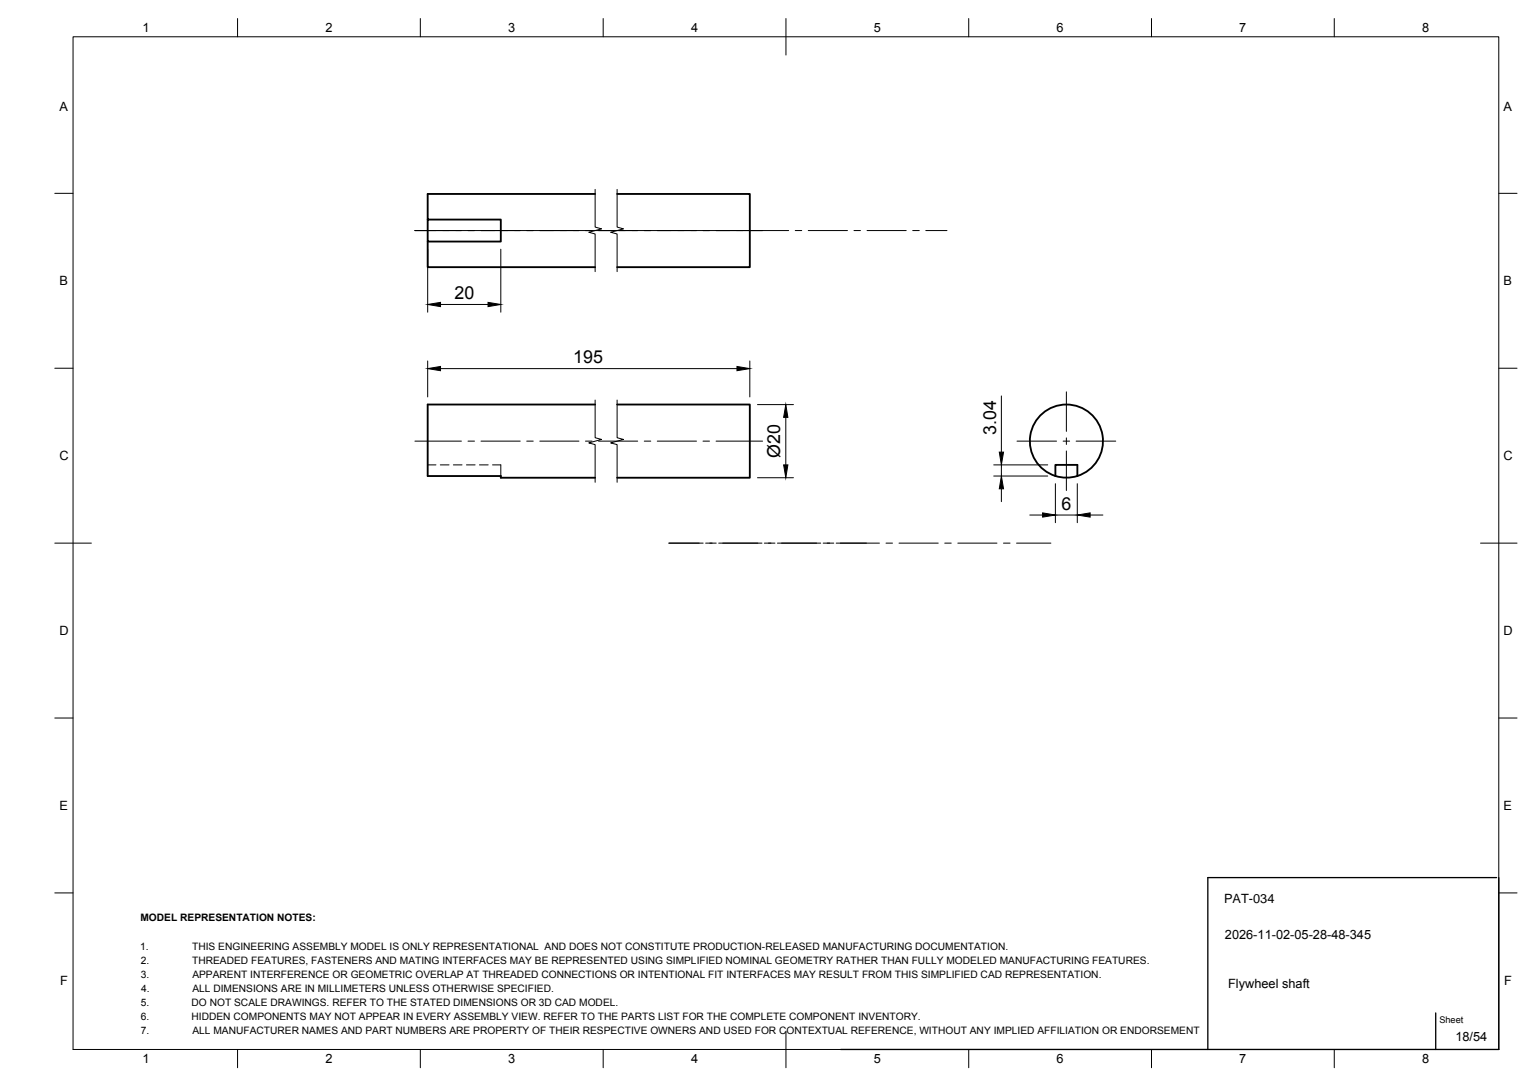
ISO-10303-21;
HEADER;
/* Generated by software containing ST-Developer
 * from STEP Tools, Inc. (www.steptools.com) 
 */

FILE_DESCRIPTION(
/* description */ ('Fatigue rig crank-slider'),
/* implementation_level */ '2;1');

FILE_NAME(
/* name */ 'Flywheel shaft.step',
/* time_stamp */ '2026-10-28T03:24:50-07:00',
/* author */ (''),
/* organization */ (''),
/* preprocessor_version */ 'ST-DEVELOPER v20.2',
/* originating_system */ 'Autodesk Translation Framework v15.17.0.0',
/* authorisation */ '');

FILE_SCHEMA (('AUTOMOTIVE_DESIGN { 1 0 10303 214 3 1 1 }'));
ENDSEC;

DATA;
#10=MECHANICAL_DESIGN_GEOMETRIC_PRESENTATION_REPRESENTATION('',(#604),#16911);
#503=SHAPE_REPRESENTATION_RELATIONSHIP('SRR','None',#17144,#553);
#553=ADVANCED_BREP_SHAPE_REPRESENTATION('',(#661),#16873);
#604=STYLED_ITEM('',(#17487),#661);
#661=MANIFOLD_SOLID_BREP('Body1',#8897);
#1027=PLANE('',#9901);
#1028=PLANE('',#9902);
#1029=PLANE('',#9904);
#1030=PLANE('',#9905);
#1031=PLANE('',#9910);
#1032=PLANE('',#9911);
#1437=FACE_OUTER_BOUND('',#2081,.T.);
#1438=FACE_OUTER_BOUND('',#2082,.T.);
#1439=FACE_OUTER_BOUND('',#2083,.T.);
#1440=FACE_OUTER_BOUND('',#2084,.T.);
#1441=FACE_OUTER_BOUND('',#2085,.T.);
#1442=FACE_OUTER_BOUND('',#2086,.T.);
#1443=FACE_OUTER_BOUND('',#2087,.T.);
#2081=EDGE_LOOP('',(#6920,#6921,#6922,#6923));
#2082=EDGE_LOOP('',(#6924,#6925,#6926,#6927));
#2083=EDGE_LOOP('',(#6928,#6929,#6930,#6931));
#2084=EDGE_LOOP('',(#6932,#6933,#6934,#6935));
#2085=EDGE_LOOP('',(#6936,#6937,#6938,#6939,#6940,#6941,#6942,#6943));
#2086=EDGE_LOOP('',(#6944,#6945,#6946,#6947,#6948));
#2087=EDGE_LOOP('',(#6949));
#2733=LINE('',#14787,#3379);
#2734=LINE('',#14789,#3380);
#2735=LINE('',#14791,#3381);
#2736=LINE('',#14792,#3382);
#2737=LINE('',#14797,#3383);
#2738=LINE('',#14798,#3384);
#2739=LINE('',#14801,#3385);
#2740=LINE('',#14803,#3386);
#2741=LINE('',#14804,#3387);
#2742=LINE('',#14806,#3388);
#2743=LINE('',#14811,#3389);
#3379=VECTOR('',#11657,1.);
#3380=VECTOR('',#11658,1.);
#3381=VECTOR('',#11659,1.);
#3382=VECTOR('',#11660,1.);
#3383=VECTOR('',#11665,1.);
#3384=VECTOR('',#11666,1.);
#3385=VECTOR('',#11669,1.);
#3386=VECTOR('',#11670,1.);
#3387=VECTOR('',#11671,1.);
#3388=VECTOR('',#11674,1.);
#3389=VECTOR('',#11679,1.);
#3917=CIRCLE('',#9903,1.);
#3918=CIRCLE('',#9907,1.);
#3919=CIRCLE('',#9908,1.);
#3920=CIRCLE('',#9909,1.);
#4465=VERTEX_POINT('',#14785);
#4466=VERTEX_POINT('',#14786);
#4467=VERTEX_POINT('',#14788);
#4468=VERTEX_POINT('',#14790);
#4469=VERTEX_POINT('',#14794);
#4470=VERTEX_POINT('',#14796);
#4471=VERTEX_POINT('',#14800);
#4472=VERTEX_POINT('',#14802);
#4473=VERTEX_POINT('',#14808);
#4474=VERTEX_POINT('',#14810);
#5358=EDGE_CURVE('',#4465,#4466,#2733,.T.);
#5359=EDGE_CURVE('',#4467,#4465,#2734,.T.);
#5360=EDGE_CURVE('',#4468,#4467,#2735,.T.);
#5361=EDGE_CURVE('',#4468,#4466,#2736,.T.);
#5362=EDGE_CURVE('',#4466,#4469,#3917,.T.);
#5363=EDGE_CURVE('',#4470,#4468,#2737,.T.);
#5364=EDGE_CURVE('',#4469,#4470,#2738,.T.);
#5365=EDGE_CURVE('',#4469,#4471,#2739,.T.);
#5366=EDGE_CURVE('',#4470,#4472,#2740,.T.);
#5367=EDGE_CURVE('',#4471,#4472,#2741,.T.);
#5368=EDGE_CURVE('',#4472,#4467,#2742,.T.);
#5369=EDGE_CURVE('',#4473,#4471,#3918,.T.);
#5370=EDGE_CURVE('',#4473,#4474,#2743,.T.);
#5371=EDGE_CURVE('',#4474,#4474,#3919,.T.);
#5372=EDGE_CURVE('',#4465,#4473,#3920,.T.);
#6920=ORIENTED_EDGE('',*,*,#5358,.F.);
#6921=ORIENTED_EDGE('',*,*,#5359,.F.);
#6922=ORIENTED_EDGE('',*,*,#5360,.F.);
#6923=ORIENTED_EDGE('',*,*,#5361,.T.);
#6924=ORIENTED_EDGE('',*,*,#5362,.F.);
#6925=ORIENTED_EDGE('',*,*,#5361,.F.);
#6926=ORIENTED_EDGE('',*,*,#5363,.F.);
#6927=ORIENTED_EDGE('',*,*,#5364,.F.);
#6928=ORIENTED_EDGE('',*,*,#5365,.F.);
#6929=ORIENTED_EDGE('',*,*,#5364,.T.);
#6930=ORIENTED_EDGE('',*,*,#5366,.T.);
#6931=ORIENTED_EDGE('',*,*,#5367,.F.);
#6932=ORIENTED_EDGE('',*,*,#5363,.T.);
#6933=ORIENTED_EDGE('',*,*,#5360,.T.);
#6934=ORIENTED_EDGE('',*,*,#5368,.F.);
#6935=ORIENTED_EDGE('',*,*,#5366,.F.);
#6936=ORIENTED_EDGE('',*,*,#5358,.T.);
#6937=ORIENTED_EDGE('',*,*,#5362,.T.);
#6938=ORIENTED_EDGE('',*,*,#5365,.T.);
#6939=ORIENTED_EDGE('',*,*,#5369,.F.);
#6940=ORIENTED_EDGE('',*,*,#5370,.T.);
#6941=ORIENTED_EDGE('',*,*,#5371,.T.);
#6942=ORIENTED_EDGE('',*,*,#5370,.F.);
#6943=ORIENTED_EDGE('',*,*,#5372,.F.);
#6944=ORIENTED_EDGE('',*,*,#5359,.T.);
#6945=ORIENTED_EDGE('',*,*,#5372,.T.);
#6946=ORIENTED_EDGE('',*,*,#5369,.T.);
#6947=ORIENTED_EDGE('',*,*,#5367,.T.);
#6948=ORIENTED_EDGE('',*,*,#5368,.T.);
#6949=ORIENTED_EDGE('',*,*,#5371,.F.);
#8277=CYLINDRICAL_SURFACE('',#9906,1.);
#8575=ADVANCED_FACE('',(#1437),#1027,.F.);
#8576=ADVANCED_FACE('',(#1438),#1028,.T.);
#8577=ADVANCED_FACE('',(#1439),#1029,.F.);
#8578=ADVANCED_FACE('',(#1440),#1030,.F.);
#8579=ADVANCED_FACE('',(#1441),#8277,.T.);
#8580=ADVANCED_FACE('',(#1442),#1031,.T.);
#8581=ADVANCED_FACE('',(#1443),#1032,.F.);
#8897=CLOSED_SHELL('',(#8575,#8576,#8577,#8578,#8579,#8580,#8581));
#9900=AXIS2_PLACEMENT_3D('',#14783,#11653,#11654);
#9901=AXIS2_PLACEMENT_3D('',#14784,#11655,#11656);
#9902=AXIS2_PLACEMENT_3D('',#14793,#11661,#11662);
#9903=AXIS2_PLACEMENT_3D('',#14795,#11663,#11664);
#9904=AXIS2_PLACEMENT_3D('',#14799,#11667,#11668);
#9905=AXIS2_PLACEMENT_3D('',#14805,#11672,#11673);
#9906=AXIS2_PLACEMENT_3D('',#14807,#11675,#11676);
#9907=AXIS2_PLACEMENT_3D('',#14809,#11677,#11678);
#9908=AXIS2_PLACEMENT_3D('',#14812,#11680,#11681);
#9909=AXIS2_PLACEMENT_3D('',#14813,#11682,#11683);
#9910=AXIS2_PLACEMENT_3D('',#14814,#11684,#11685);
#9911=AXIS2_PLACEMENT_3D('',#14815,#11686,#11687);
#11653=DIRECTION('axis',(0.,0.,1.));
#11654=DIRECTION('refdir',(1.,0.,0.));
#11655=DIRECTION('center_axis',(-1.,0.,0.));
#11656=DIRECTION('ref_axis',(0.,0.,1.));
#11657=DIRECTION('',(0.,-1.,0.));
#11658=DIRECTION('',(0.,0.,-1.));
#11659=DIRECTION('',(0.,1.,0.));
#11660=DIRECTION('',(0.,0.,-1.));
#11661=DIRECTION('center_axis',(0.,1.,0.));
#11662=DIRECTION('ref_axis',(1.,0.,0.));
#11663=DIRECTION('center_axis',(0.,-1.,0.));
#11664=DIRECTION('ref_axis',(1.,0.,0.));
#11665=DIRECTION('',(-1.,0.,0.));
#11666=DIRECTION('',(0.,0.,1.));
#11667=DIRECTION('center_axis',(1.,0.,0.));
#11668=DIRECTION('ref_axis',(0.,0.,-1.));
#11669=DIRECTION('',(0.,1.,0.));
#11670=DIRECTION('',(0.,1.,0.));
#11671=DIRECTION('',(0.,0.,1.));
#11672=DIRECTION('center_axis',(0.,0.,1.));
#11673=DIRECTION('ref_axis',(1.,0.,0.));
#11674=DIRECTION('',(-1.,0.,0.));
#11675=DIRECTION('center_axis',(0.,1.,0.));
#11676=DIRECTION('ref_axis',(1.,0.,0.));
#11677=DIRECTION('center_axis',(0.,1.,0.));
#11678=DIRECTION('ref_axis',(1.,0.,0.));
#11679=DIRECTION('',(0.,-1.,0.));
#11680=DIRECTION('center_axis',(0.,1.,0.));
#11681=DIRECTION('ref_axis',(1.,0.,0.));
#11682=DIRECTION('center_axis',(0.,1.,0.));
#11683=DIRECTION('ref_axis',(1.,0.,0.));
#11684=DIRECTION('center_axis',(0.,1.,0.));
#11685=DIRECTION('ref_axis',(1.,0.,0.));
#11686=DIRECTION('center_axis',(0.,1.,0.));
#11687=DIRECTION('ref_axis',(1.,0.,0.));
#14783=CARTESIAN_POINT('',(0.,0.,0.));
#14784=CARTESIAN_POINT('Origin',(-0.3,-1.5,10.9));
#14785=CARTESIAN_POINT('',(-0.3,0.5,11.0460607985831));
#14786=CARTESIAN_POINT('',(-0.3,-1.5,11.0460607985831));
#14787=CARTESIAN_POINT('',(-0.3,-19.,11.0460607985831));
#14788=CARTESIAN_POINT('',(-0.3,0.5,11.35));
#14789=CARTESIAN_POINT('',(-0.3,0.5,11.45));
#14790=CARTESIAN_POINT('',(-0.3,-1.5,11.35));
#14791=CARTESIAN_POINT('',(-0.3,-1.5,11.35));
#14792=CARTESIAN_POINT('',(-0.3,-1.5,11.35));
#14793=CARTESIAN_POINT('Origin',(0.,-1.5,11.125));
#14794=CARTESIAN_POINT('',(0.3,-1.5,11.0460607985831));
#14795=CARTESIAN_POINT('Origin',(0.,-1.5,12.));
#14796=CARTESIAN_POINT('',(0.3,-1.5,11.35));
#14797=CARTESIAN_POINT('',(0.3,-1.5,11.35));
#14798=CARTESIAN_POINT('',(0.3,-1.5,10.9));
#14799=CARTESIAN_POINT('Origin',(0.3,-1.5,11.35));
#14800=CARTESIAN_POINT('',(0.3,0.5,11.0460607985831));
#14801=CARTESIAN_POINT('',(0.3,-19.,11.0460607985831));
#14802=CARTESIAN_POINT('',(0.3,0.5,11.35));
#14803=CARTESIAN_POINT('',(0.3,-1.5,11.35));
#14804=CARTESIAN_POINT('',(0.3,0.5,11.675));
#14805=CARTESIAN_POINT('Origin',(-0.3,-1.5,11.35));
#14806=CARTESIAN_POINT('',(-0.15,0.5,11.35));
#14807=CARTESIAN_POINT('Origin',(0.,-19.,12.));
#14808=CARTESIAN_POINT('',(-1.,0.5,12.));
#14809=CARTESIAN_POINT('Origin',(0.,0.5,12.));
#14810=CARTESIAN_POINT('',(-1.,-19.,12.));
#14811=CARTESIAN_POINT('',(-1.,-19.,12.));
#14812=CARTESIAN_POINT('Origin',(0.,-19.,12.));
#14813=CARTESIAN_POINT('Origin',(0.,0.5,12.));
#14814=CARTESIAN_POINT('Origin',(0.,0.5,12.));
#14815=CARTESIAN_POINT('Origin',(0.,-19.,12.));
#16814=UNCERTAINTY_MEASURE_WITH_UNIT(LENGTH_MEASURE(0.001),#16912,
'DISTANCE_ACCURACY_VALUE',
'Maximum model space distance between geometric entities at asserted c
onnectivities');
#16852=UNCERTAINTY_MEASURE_WITH_UNIT(LENGTH_MEASURE(0.001),#16912,
'DISTANCE_ACCURACY_VALUE',
'Maximum model space distance between geometric entities at asserted c
onnectivities');
#16873=(
GEOMETRIC_REPRESENTATION_CONTEXT(3)
GLOBAL_UNCERTAINTY_ASSIGNED_CONTEXT((#16814))
GLOBAL_UNIT_ASSIGNED_CONTEXT((#16912,#16914,#16915))
REPRESENTATION_CONTEXT('','3D')
);
#16911=(
GEOMETRIC_REPRESENTATION_CONTEXT(3)
GLOBAL_UNCERTAINTY_ASSIGNED_CONTEXT((#16852))
GLOBAL_UNIT_ASSIGNED_CONTEXT((#16912,#16914,#16915))
REPRESENTATION_CONTEXT('','3D')
);
#16912=(
LENGTH_UNIT()
NAMED_UNIT(*)
SI_UNIT(.CENTI.,.METRE.)
);
#16914=(
NAMED_UNIT(*)
PLANE_ANGLE_UNIT()
SI_UNIT($,.RADIAN.)
);
#16915=(
NAMED_UNIT(*)
SI_UNIT($,.STERADIAN.)
SOLID_ANGLE_UNIT()
);
#16936=SHAPE_DEFINITION_REPRESENTATION(#16996,#17144);
#16996=PRODUCT_DEFINITION_SHAPE('',$,#17203);
#17144=SHAPE_REPRESENTATION('',(#9900),#16873);
#17182=PRODUCT_DEFINITION_CONTEXT('part definition',#17358,'design');
#17203=PRODUCT_DEFINITION('Flywheel shaft','Flywheel shaft',#17261,#17182);
#17261=PRODUCT_DEFINITION_FORMATION('',$,#17380);
#17358=APPLICATION_CONTEXT(
'Core Data for Automotive Mechanical Design Process');
#17359=PRODUCT_CONTEXT('part definition',#17358,'mechanical');
#17380=PRODUCT('Flywheel shaft','Flywheel shaft','Flywheel shaft',(#17359));
#17481=COLOUR_RGB('Grey',0.48,0.52,0.57);
#17482=FILL_AREA_STYLE_COLOUR('',#17481);
#17483=FILL_AREA_STYLE('',(#17482));
#17484=SURFACE_STYLE_FILL_AREA(#17483);
#17485=SURFACE_SIDE_STYLE('',(#17484));
#17486=SURFACE_STYLE_USAGE(.BOTH.,#17485);
#17487=PRESENTATION_STYLE_ASSIGNMENT((#17486));
ENDSEC;
END-ISO-10303-21;
